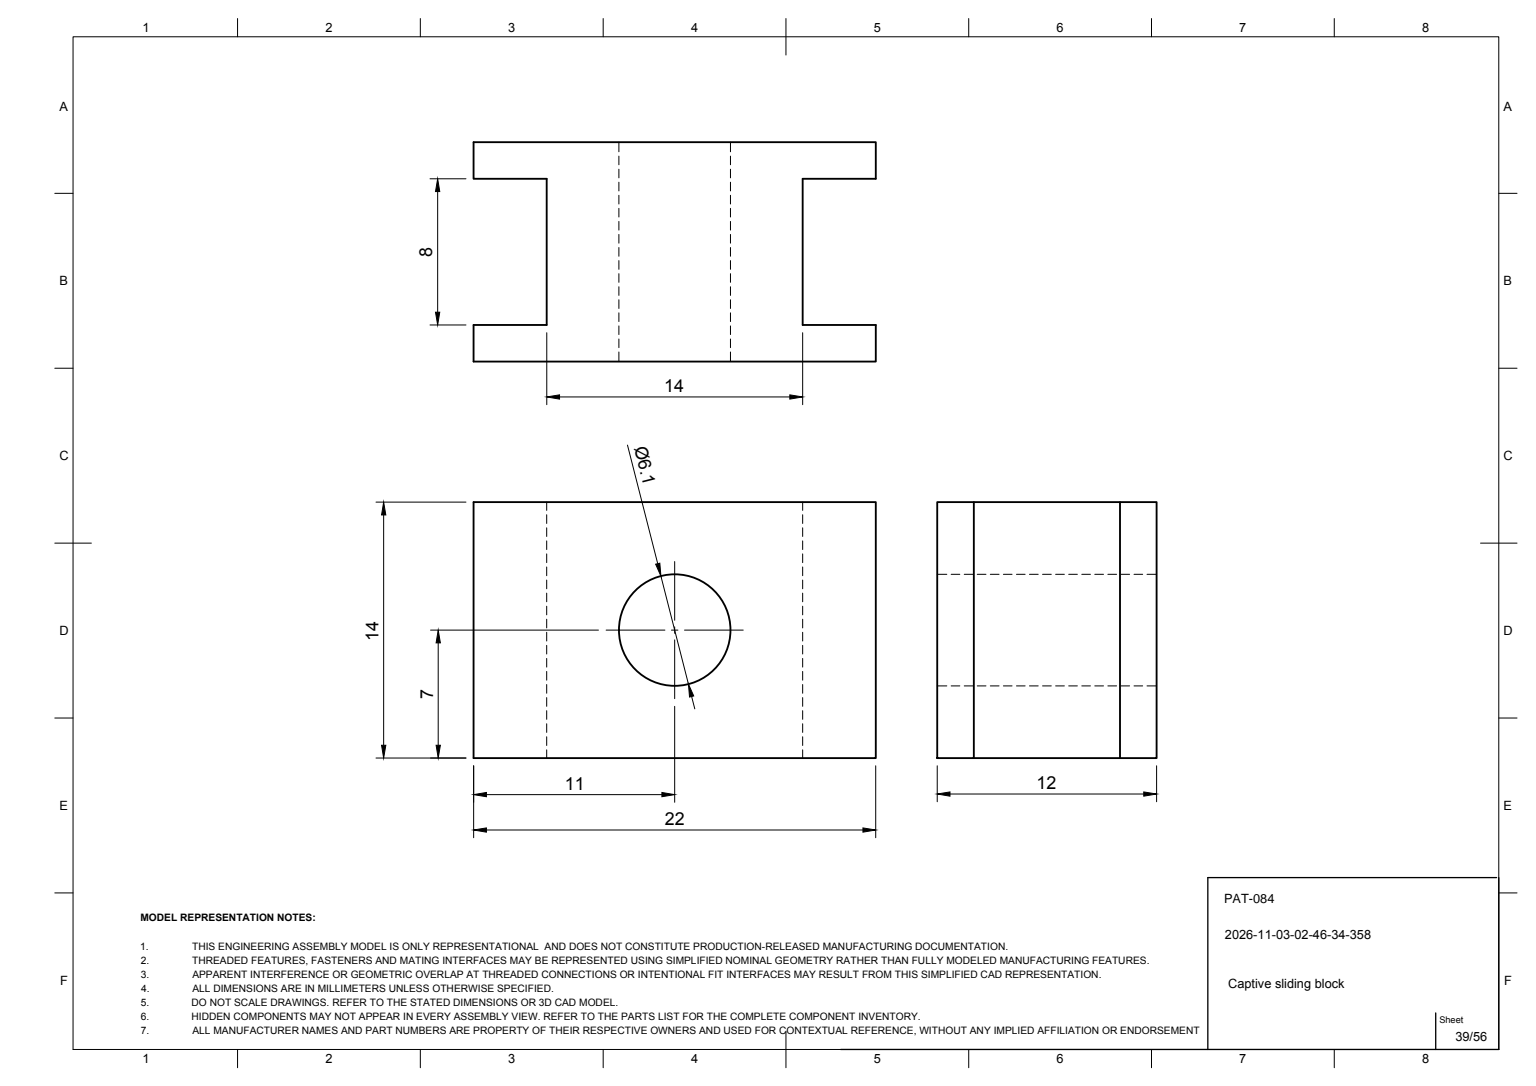
ISO-10303-21;
HEADER;
/* Generated by software containing ST-Developer
 * from STEP Tools, Inc. (www.steptools.com) 
 */

FILE_DESCRIPTION(
/* description */ ('Quick-return (Whitworth) mechanism'),
/* implementation_level */ '2;1');

FILE_NAME(
/* name */ 'Captive sliding block.step',
/* time_stamp */ '2026-10-28T03:25:57-07:00',
/* author */ (''),
/* organization */ (''),
/* preprocessor_version */ 'ST-DEVELOPER v20.2',
/* originating_system */ 'Autodesk Translation Framework v15.17.0.0',
/* authorisation */ '');

FILE_SCHEMA (('AUTOMOTIVE_DESIGN { 1 0 10303 214 3 1 1 }'));
ENDSEC;

DATA;
#10=MECHANICAL_DESIGN_GEOMETRIC_PRESENTATION_REPRESENTATION('',(#528),#14878);
#432=SHAPE_REPRESENTATION_RELATIONSHIP('SRR','None',#15104,#476);
#476=ADVANCED_BREP_SHAPE_REPRESENTATION('',(#579),#14861);
#528=STYLED_ITEM('',(#15385),#579);
#579=MANIFOLD_SOLID_BREP('Body1',#7883);
#747=FACE_BOUND('',#2004,.T.);
#748=FACE_BOUND('',#2010,.T.);
#948=PLANE('',#9095);
#949=PLANE('',#9096);
#950=PLANE('',#9097);
#951=PLANE('',#9098);
#952=PLANE('',#9099);
#953=PLANE('',#9100);
#954=PLANE('',#9101);
#955=PLANE('',#9102);
#956=PLANE('',#9103);
#957=PLANE('',#9104);
#958=PLANE('',#9105);
#959=PLANE('',#9106);
#960=PLANE('',#9107);
#961=PLANE('',#9108);
#1376=FACE_OUTER_BOUND('',#1998,.T.);
#1377=FACE_OUTER_BOUND('',#1999,.T.);
#1378=FACE_OUTER_BOUND('',#2000,.T.);
#1379=FACE_OUTER_BOUND('',#2001,.T.);
#1380=FACE_OUTER_BOUND('',#2002,.T.);
#1381=FACE_OUTER_BOUND('',#2003,.T.);
#1382=FACE_OUTER_BOUND('',#2005,.T.);
#1383=FACE_OUTER_BOUND('',#2006,.T.);
#1384=FACE_OUTER_BOUND('',#2007,.T.);
#1385=FACE_OUTER_BOUND('',#2008,.T.);
#1386=FACE_OUTER_BOUND('',#2009,.T.);
#1387=FACE_OUTER_BOUND('',#2011,.T.);
#1388=FACE_OUTER_BOUND('',#2012,.T.);
#1389=FACE_OUTER_BOUND('',#2013,.T.);
#1390=FACE_OUTER_BOUND('',#2014,.T.);
#1998=EDGE_LOOP('',(#6598,#6599,#6600,#6601));
#1999=EDGE_LOOP('',(#6602,#6603,#6604,#6605));
#2000=EDGE_LOOP('',(#6606,#6607,#6608,#6609));
#2001=EDGE_LOOP('',(#6610,#6611,#6612,#6613));
#2002=EDGE_LOOP('',(#6614,#6615,#6616,#6617));
#2003=EDGE_LOOP('',(#6618,#6619,#6620,#6621));
#2004=EDGE_LOOP('',(#6622));
#2005=EDGE_LOOP('',(#6623,#6624,#6625,#6626));
#2006=EDGE_LOOP('',(#6627,#6628,#6629,#6630));
#2007=EDGE_LOOP('',(#6631,#6632,#6633,#6634));
#2008=EDGE_LOOP('',(#6635,#6636,#6637,#6638));
#2009=EDGE_LOOP('',(#6639,#6640,#6641,#6642));
#2010=EDGE_LOOP('',(#6643));
#2011=EDGE_LOOP('',(#6644,#6645,#6646,#6647,#6648,#6649,#6650,#6651,#6652,
#6653,#6654,#6655));
#2012=EDGE_LOOP('',(#6656,#6657,#6658,#6659));
#2013=EDGE_LOOP('',(#6660,#6661,#6662,#6663,#6664,#6665,#6666,#6667,#6668,
#6669,#6670,#6671));
#2014=EDGE_LOOP('',(#6672,#6673,#6674,#6675));
#2465=LINE('',#14040,#2988);
#2466=LINE('',#14045,#2989);
#2467=LINE('',#14047,#2990);
#2468=LINE('',#14049,#2991);
#2469=LINE('',#14050,#2992);
#2470=LINE('',#14054,#2993);
#2471=LINE('',#14056,#2994);
#2472=LINE('',#14058,#2995);
#2473=LINE('',#14059,#2996);
#2474=LINE('',#14062,#2997);
#2475=LINE('',#14064,#2998);
#2476=LINE('',#14065,#2999);
#2477=LINE('',#14068,#3000);
#2478=LINE('',#14070,#3001);
#2479=LINE('',#14071,#3002);
#2480=LINE('',#14073,#3003);
#2481=LINE('',#14074,#3004);
#2482=LINE('',#14078,#3005);
#2483=LINE('',#14080,#3006);
#2484=LINE('',#14082,#3007);
#2485=LINE('',#14083,#3008);
#2486=LINE('',#14087,#3009);
#2487=LINE('',#14089,#3010);
#2488=LINE('',#14091,#3011);
#2489=LINE('',#14092,#3012);
#2490=LINE('',#14096,#3013);
#2491=LINE('',#14097,#3014);
#2492=LINE('',#14098,#3015);
#2493=LINE('',#14102,#3016);
#2494=LINE('',#14103,#3017);
#2495=LINE('',#14104,#3018);
#2496=LINE('',#14106,#3019);
#2497=LINE('',#14107,#3020);
#2498=LINE('',#14109,#3021);
#2499=LINE('',#14110,#3022);
#2500=LINE('',#14112,#3023);
#2501=LINE('',#14114,#3024);
#2988=VECTOR('',#11112,0.305);
#2989=VECTOR('',#11117,1.);
#2990=VECTOR('',#11118,1.);
#2991=VECTOR('',#11119,1.);
#2992=VECTOR('',#11120,1.);
#2993=VECTOR('',#11123,1.);
#2994=VECTOR('',#11124,1.);
#2995=VECTOR('',#11125,1.);
#2996=VECTOR('',#11126,1.);
#2997=VECTOR('',#11129,1.);
#2998=VECTOR('',#11130,1.);
#2999=VECTOR('',#11131,1.);
#3000=VECTOR('',#11134,1.);
#3001=VECTOR('',#11135,1.);
#3002=VECTOR('',#11136,1.);
#3003=VECTOR('',#11139,1.);
#3004=VECTOR('',#11140,1.);
#3005=VECTOR('',#11143,1.);
#3006=VECTOR('',#11144,1.);
#3007=VECTOR('',#11145,1.);
#3008=VECTOR('',#11146,1.);
#3009=VECTOR('',#11149,1.);
#3010=VECTOR('',#11150,1.);
#3011=VECTOR('',#11151,1.);
#3012=VECTOR('',#11152,1.);
#3013=VECTOR('',#11155,1.);
#3014=VECTOR('',#11156,1.);
#3015=VECTOR('',#11157,1.);
#3016=VECTOR('',#11160,1.);
#3017=VECTOR('',#11161,1.);
#3018=VECTOR('',#11162,1.);
#3019=VECTOR('',#11165,1.);
#3020=VECTOR('',#11166,1.);
#3021=VECTOR('',#11169,1.);
#3022=VECTOR('',#11170,1.);
#3023=VECTOR('',#11173,1.);
#3024=VECTOR('',#11176,1.);
#3553=CIRCLE('',#9093,0.305);
#3554=CIRCLE('',#9094,0.305);
#4086=VERTEX_POINT('',#14037);
#4087=VERTEX_POINT('',#14039);
#4088=VERTEX_POINT('',#14043);
#4089=VERTEX_POINT('',#14044);
#4090=VERTEX_POINT('',#14046);
#4091=VERTEX_POINT('',#14048);
#4092=VERTEX_POINT('',#14052);
#4093=VERTEX_POINT('',#14053);
#4094=VERTEX_POINT('',#14055);
#4095=VERTEX_POINT('',#14057);
#4096=VERTEX_POINT('',#14061);
#4097=VERTEX_POINT('',#14063);
#4098=VERTEX_POINT('',#14067);
#4099=VERTEX_POINT('',#14069);
#4100=VERTEX_POINT('',#14076);
#4101=VERTEX_POINT('',#14077);
#4102=VERTEX_POINT('',#14079);
#4103=VERTEX_POINT('',#14081);
#4104=VERTEX_POINT('',#14085);
#4105=VERTEX_POINT('',#14086);
#4106=VERTEX_POINT('',#14088);
#4107=VERTEX_POINT('',#14090);
#4108=VERTEX_POINT('',#14094);
#4109=VERTEX_POINT('',#14095);
#4110=VERTEX_POINT('',#14100);
#4111=VERTEX_POINT('',#14101);
#4956=EDGE_CURVE('',#4086,#4086,#3553,.T.);
#4957=EDGE_CURVE('',#4086,#4087,#2465,.T.);
#4958=EDGE_CURVE('',#4087,#4087,#3554,.T.);
#4959=EDGE_CURVE('',#4088,#4089,#2466,.T.);
#4960=EDGE_CURVE('',#4090,#4089,#2467,.T.);
#4961=EDGE_CURVE('',#4091,#4090,#2468,.T.);
#4962=EDGE_CURVE('',#4088,#4091,#2469,.T.);
#4963=EDGE_CURVE('',#4092,#4093,#2470,.T.);
#4964=EDGE_CURVE('',#4094,#4093,#2471,.T.);
#4965=EDGE_CURVE('',#4095,#4094,#2472,.T.);
#4966=EDGE_CURVE('',#4092,#4095,#2473,.T.);
#4967=EDGE_CURVE('',#4090,#4096,#2474,.T.);
#4968=EDGE_CURVE('',#4097,#4096,#2475,.T.);
#4969=EDGE_CURVE('',#4091,#4097,#2476,.T.);
#4970=EDGE_CURVE('',#4094,#4098,#2477,.T.);
#4971=EDGE_CURVE('',#4099,#4098,#2478,.T.);
#4972=EDGE_CURVE('',#4095,#4099,#2479,.T.);
#4973=EDGE_CURVE('',#4098,#4097,#2480,.T.);
#4974=EDGE_CURVE('',#4096,#4099,#2481,.T.);
#4975=EDGE_CURVE('',#4100,#4101,#2482,.T.);
#4976=EDGE_CURVE('',#4100,#4102,#2483,.T.);
#4977=EDGE_CURVE('',#4102,#4103,#2484,.T.);
#4978=EDGE_CURVE('',#4103,#4101,#2485,.T.);
#4979=EDGE_CURVE('',#4104,#4105,#2486,.T.);
#4980=EDGE_CURVE('',#4104,#4106,#2487,.T.);
#4981=EDGE_CURVE('',#4106,#4107,#2488,.T.);
#4982=EDGE_CURVE('',#4107,#4105,#2489,.T.);
#4983=EDGE_CURVE('',#4108,#4109,#2490,.T.);
#4984=EDGE_CURVE('',#4109,#4107,#2491,.T.);
#4985=EDGE_CURVE('',#4108,#4106,#2492,.T.);
#4986=EDGE_CURVE('',#4110,#4111,#2493,.T.);
#4987=EDGE_CURVE('',#4111,#4103,#2494,.T.);
#4988=EDGE_CURVE('',#4110,#4102,#2495,.T.);
#4989=EDGE_CURVE('',#4109,#4110,#2496,.T.);
#4990=EDGE_CURVE('',#4111,#4108,#2497,.T.);
#4991=EDGE_CURVE('',#4100,#4092,#2498,.T.);
#4992=EDGE_CURVE('',#4105,#4089,#2499,.T.);
#4993=EDGE_CURVE('',#4104,#4088,#2500,.T.);
#4994=EDGE_CURVE('',#4101,#4093,#2501,.T.);
#6598=ORIENTED_EDGE('',*,*,#4956,.F.);
#6599=ORIENTED_EDGE('',*,*,#4957,.T.);
#6600=ORIENTED_EDGE('',*,*,#4958,.F.);
#6601=ORIENTED_EDGE('',*,*,#4957,.F.);
#6602=ORIENTED_EDGE('',*,*,#4959,.T.);
#6603=ORIENTED_EDGE('',*,*,#4960,.F.);
#6604=ORIENTED_EDGE('',*,*,#4961,.F.);
#6605=ORIENTED_EDGE('',*,*,#4962,.F.);
#6606=ORIENTED_EDGE('',*,*,#4963,.T.);
#6607=ORIENTED_EDGE('',*,*,#4964,.F.);
#6608=ORIENTED_EDGE('',*,*,#4965,.F.);
#6609=ORIENTED_EDGE('',*,*,#4966,.F.);
#6610=ORIENTED_EDGE('',*,*,#4961,.T.);
#6611=ORIENTED_EDGE('',*,*,#4967,.T.);
#6612=ORIENTED_EDGE('',*,*,#4968,.F.);
#6613=ORIENTED_EDGE('',*,*,#4969,.F.);
#6614=ORIENTED_EDGE('',*,*,#4965,.T.);
#6615=ORIENTED_EDGE('',*,*,#4970,.T.);
#6616=ORIENTED_EDGE('',*,*,#4971,.F.);
#6617=ORIENTED_EDGE('',*,*,#4972,.F.);
#6618=ORIENTED_EDGE('',*,*,#4971,.T.);
#6619=ORIENTED_EDGE('',*,*,#4973,.T.);
#6620=ORIENTED_EDGE('',*,*,#4968,.T.);
#6621=ORIENTED_EDGE('',*,*,#4974,.T.);
#6622=ORIENTED_EDGE('',*,*,#4958,.T.);
#6623=ORIENTED_EDGE('',*,*,#4975,.F.);
#6624=ORIENTED_EDGE('',*,*,#4976,.T.);
#6625=ORIENTED_EDGE('',*,*,#4977,.T.);
#6626=ORIENTED_EDGE('',*,*,#4978,.T.);
#6627=ORIENTED_EDGE('',*,*,#4979,.F.);
#6628=ORIENTED_EDGE('',*,*,#4980,.T.);
#6629=ORIENTED_EDGE('',*,*,#4981,.T.);
#6630=ORIENTED_EDGE('',*,*,#4982,.T.);
#6631=ORIENTED_EDGE('',*,*,#4983,.T.);
#6632=ORIENTED_EDGE('',*,*,#4984,.T.);
#6633=ORIENTED_EDGE('',*,*,#4981,.F.);
#6634=ORIENTED_EDGE('',*,*,#4985,.F.);
#6635=ORIENTED_EDGE('',*,*,#4986,.T.);
#6636=ORIENTED_EDGE('',*,*,#4987,.T.);
#6637=ORIENTED_EDGE('',*,*,#4977,.F.);
#6638=ORIENTED_EDGE('',*,*,#4988,.F.);
#6639=ORIENTED_EDGE('',*,*,#4986,.F.);
#6640=ORIENTED_EDGE('',*,*,#4989,.F.);
#6641=ORIENTED_EDGE('',*,*,#4983,.F.);
#6642=ORIENTED_EDGE('',*,*,#4990,.F.);
#6643=ORIENTED_EDGE('',*,*,#4956,.T.);
#6644=ORIENTED_EDGE('',*,*,#4991,.T.);
#6645=ORIENTED_EDGE('',*,*,#4966,.T.);
#6646=ORIENTED_EDGE('',*,*,#4972,.T.);
#6647=ORIENTED_EDGE('',*,*,#4974,.F.);
#6648=ORIENTED_EDGE('',*,*,#4967,.F.);
#6649=ORIENTED_EDGE('',*,*,#4960,.T.);
#6650=ORIENTED_EDGE('',*,*,#4992,.F.);
#6651=ORIENTED_EDGE('',*,*,#4982,.F.);
#6652=ORIENTED_EDGE('',*,*,#4984,.F.);
#6653=ORIENTED_EDGE('',*,*,#4989,.T.);
#6654=ORIENTED_EDGE('',*,*,#4988,.T.);
#6655=ORIENTED_EDGE('',*,*,#4976,.F.);
#6656=ORIENTED_EDGE('',*,*,#4979,.T.);
#6657=ORIENTED_EDGE('',*,*,#4992,.T.);
#6658=ORIENTED_EDGE('',*,*,#4959,.F.);
#6659=ORIENTED_EDGE('',*,*,#4993,.F.);
#6660=ORIENTED_EDGE('',*,*,#4993,.T.);
#6661=ORIENTED_EDGE('',*,*,#4962,.T.);
#6662=ORIENTED_EDGE('',*,*,#4969,.T.);
#6663=ORIENTED_EDGE('',*,*,#4973,.F.);
#6664=ORIENTED_EDGE('',*,*,#4970,.F.);
#6665=ORIENTED_EDGE('',*,*,#4964,.T.);
#6666=ORIENTED_EDGE('',*,*,#4994,.F.);
#6667=ORIENTED_EDGE('',*,*,#4978,.F.);
#6668=ORIENTED_EDGE('',*,*,#4987,.F.);
#6669=ORIENTED_EDGE('',*,*,#4990,.T.);
#6670=ORIENTED_EDGE('',*,*,#4985,.T.);
#6671=ORIENTED_EDGE('',*,*,#4980,.F.);
#6672=ORIENTED_EDGE('',*,*,#4975,.T.);
#6673=ORIENTED_EDGE('',*,*,#4994,.T.);
#6674=ORIENTED_EDGE('',*,*,#4963,.F.);
#6675=ORIENTED_EDGE('',*,*,#4991,.F.);
#7346=CYLINDRICAL_SURFACE('',#9092,0.305);
#7707=ADVANCED_FACE('',(#1376),#7346,.F.);
#7708=ADVANCED_FACE('',(#1377),#948,.F.);
#7709=ADVANCED_FACE('',(#1378),#949,.F.);
#7710=ADVANCED_FACE('',(#1379),#950,.T.);
#7711=ADVANCED_FACE('',(#1380),#951,.T.);
#7712=ADVANCED_FACE('',(#1381,#747),#952,.T.);
#7713=ADVANCED_FACE('',(#1382),#953,.T.);
#7714=ADVANCED_FACE('',(#1383),#954,.T.);
#7715=ADVANCED_FACE('',(#1384),#955,.T.);
#7716=ADVANCED_FACE('',(#1385),#956,.T.);
#7717=ADVANCED_FACE('',(#1386,#748),#957,.F.);
#7718=ADVANCED_FACE('',(#1387),#958,.T.);
#7719=ADVANCED_FACE('',(#1388),#959,.T.);
#7720=ADVANCED_FACE('',(#1389),#960,.T.);
#7721=ADVANCED_FACE('',(#1390),#961,.T.);
#7883=CLOSED_SHELL('',(#7707,#7708,#7709,#7710,#7711,#7712,#7713,#7714,
#7715,#7716,#7717,#7718,#7719,#7720,#7721));
#9091=AXIS2_PLACEMENT_3D('',#14035,#11106,#11107);
#9092=AXIS2_PLACEMENT_3D('',#14036,#11108,#11109);
#9093=AXIS2_PLACEMENT_3D('',#14038,#11110,#11111);
#9094=AXIS2_PLACEMENT_3D('',#14041,#11113,#11114);
#9095=AXIS2_PLACEMENT_3D('',#14042,#11115,#11116);
#9096=AXIS2_PLACEMENT_3D('',#14051,#11121,#11122);
#9097=AXIS2_PLACEMENT_3D('',#14060,#11127,#11128);
#9098=AXIS2_PLACEMENT_3D('',#14066,#11132,#11133);
#9099=AXIS2_PLACEMENT_3D('',#14072,#11137,#11138);
#9100=AXIS2_PLACEMENT_3D('',#14075,#11141,#11142);
#9101=AXIS2_PLACEMENT_3D('',#14084,#11147,#11148);
#9102=AXIS2_PLACEMENT_3D('',#14093,#11153,#11154);
#9103=AXIS2_PLACEMENT_3D('',#14099,#11158,#11159);
#9104=AXIS2_PLACEMENT_3D('',#14105,#11163,#11164);
#9105=AXIS2_PLACEMENT_3D('',#14108,#11167,#11168);
#9106=AXIS2_PLACEMENT_3D('',#14111,#11171,#11172);
#9107=AXIS2_PLACEMENT_3D('',#14113,#11174,#11175);
#9108=AXIS2_PLACEMENT_3D('',#14115,#11177,#11178);
#11106=DIRECTION('axis',(0.,0.,1.));
#11107=DIRECTION('refdir',(1.,0.,0.));
#11108=DIRECTION('center_axis',(0.,0.,1.));
#11109=DIRECTION('ref_axis',(1.,0.,0.));
#11110=DIRECTION('center_axis',(0.,0.,1.));
#11111=DIRECTION('ref_axis',(1.,0.,0.));
#11112=DIRECTION('',(0.,0.,1.));
#11113=DIRECTION('center_axis',(0.,0.,-1.));
#11114=DIRECTION('ref_axis',(1.,0.,0.));
#11115=DIRECTION('center_axis',(0.,0.,1.));
#11116=DIRECTION('ref_axis',(1.,0.,0.));
#11117=DIRECTION('',(0.,1.,0.));
#11118=DIRECTION('',(-1.,0.,0.));
#11119=DIRECTION('',(0.,1.,0.));
#11120=DIRECTION('',(1.,0.,0.));
#11121=DIRECTION('center_axis',(0.,0.,1.));
#11122=DIRECTION('ref_axis',(1.,0.,0.));
#11123=DIRECTION('',(0.,-1.,0.));
#11124=DIRECTION('',(1.,0.,0.));
#11125=DIRECTION('',(0.,-1.,0.));
#11126=DIRECTION('',(-1.,0.,0.));
#11127=DIRECTION('center_axis',(1.,0.,0.));
#11128=DIRECTION('ref_axis',(0.,1.,0.));
#11129=DIRECTION('',(0.,0.,1.));
#11130=DIRECTION('',(0.,1.,0.));
#11131=DIRECTION('',(0.,0.,1.));
#11132=DIRECTION('center_axis',(-1.,0.,0.));
#11133=DIRECTION('ref_axis',(0.,-1.,0.));
#11134=DIRECTION('',(0.,0.,1.));
#11135=DIRECTION('',(0.,-1.,0.));
#11136=DIRECTION('',(0.,0.,1.));
#11137=DIRECTION('center_axis',(0.,0.,1.));
#11138=DIRECTION('ref_axis',(1.,0.,0.));
#11139=DIRECTION('',(1.,0.,0.));
#11140=DIRECTION('',(-1.,0.,0.));
#11141=DIRECTION('center_axis',(0.,0.,1.));
#11142=DIRECTION('ref_axis',(1.,0.,0.));
#11143=DIRECTION('',(0.,-1.,0.));
#11144=DIRECTION('',(-1.,0.,0.));
#11145=DIRECTION('',(0.,-1.,0.));
#11146=DIRECTION('',(1.,0.,0.));
#11147=DIRECTION('center_axis',(0.,0.,1.));
#11148=DIRECTION('ref_axis',(1.,0.,0.));
#11149=DIRECTION('',(0.,1.,0.));
#11150=DIRECTION('',(1.,0.,0.));
#11151=DIRECTION('',(0.,1.,0.));
#11152=DIRECTION('',(-1.,0.,0.));
#11153=DIRECTION('center_axis',(1.,0.,0.));
#11154=DIRECTION('ref_axis',(0.,1.,0.));
#11155=DIRECTION('',(0.,1.,0.));
#11156=DIRECTION('',(0.,0.,1.));
#11157=DIRECTION('',(0.,0.,1.));
#11158=DIRECTION('center_axis',(-1.,0.,0.));
#11159=DIRECTION('ref_axis',(0.,-1.,0.));
#11160=DIRECTION('',(0.,-1.,0.));
#11161=DIRECTION('',(0.,0.,1.));
#11162=DIRECTION('',(0.,0.,1.));
#11163=DIRECTION('center_axis',(0.,0.,1.));
#11164=DIRECTION('ref_axis',(1.,0.,0.));
#11165=DIRECTION('',(-1.,0.,0.));
#11166=DIRECTION('',(1.,0.,0.));
#11167=DIRECTION('center_axis',(0.,1.,0.));
#11168=DIRECTION('ref_axis',(-1.,0.,0.));
#11169=DIRECTION('',(0.,0.,1.));
#11170=DIRECTION('',(0.,0.,1.));
#11171=DIRECTION('center_axis',(1.,0.,0.));
#11172=DIRECTION('ref_axis',(0.,1.,0.));
#11173=DIRECTION('',(0.,0.,1.));
#11174=DIRECTION('center_axis',(0.,-1.,0.));
#11175=DIRECTION('ref_axis',(1.,0.,0.));
#11176=DIRECTION('',(0.,0.,1.));
#11177=DIRECTION('center_axis',(-1.,0.,0.));
#11178=DIRECTION('ref_axis',(0.,-1.,0.));
#14035=CARTESIAN_POINT('',(0.,0.,0.));
#14036=CARTESIAN_POINT('Origin',(0.,9.,6.1));
#14037=CARTESIAN_POINT('',(-0.305,9.,6.2));
#14038=CARTESIAN_POINT('Origin',(0.,9.,6.2));
#14039=CARTESIAN_POINT('',(-0.305,9.,7.4));
#14040=CARTESIAN_POINT('',(-0.305,9.,6.1));
#14041=CARTESIAN_POINT('Origin',(0.,9.,7.4));
#14042=CARTESIAN_POINT('Origin',(0.,9.,7.2));
#14043=CARTESIAN_POINT('',(0.7,8.3,7.2));
#14044=CARTESIAN_POINT('',(0.7,9.7,7.2));
#14045=CARTESIAN_POINT('',(0.7,8.3,7.2));
#14046=CARTESIAN_POINT('',(1.1,9.7,7.2));
#14047=CARTESIAN_POINT('',(1.1,9.7,7.2));
#14048=CARTESIAN_POINT('',(1.1,8.3,7.2));
#14049=CARTESIAN_POINT('',(1.1,8.3,7.2));
#14050=CARTESIAN_POINT('',(-1.1,8.3,7.2));
#14051=CARTESIAN_POINT('Origin',(0.,9.,7.2));
#14052=CARTESIAN_POINT('',(-0.7,9.7,7.2));
#14053=CARTESIAN_POINT('',(-0.7,8.3,7.2));
#14054=CARTESIAN_POINT('',(-0.7,9.7,7.2));
#14055=CARTESIAN_POINT('',(-1.1,8.3,7.2));
#14056=CARTESIAN_POINT('',(-1.1,8.3,7.2));
#14057=CARTESIAN_POINT('',(-1.1,9.7,7.2));
#14058=CARTESIAN_POINT('',(-1.1,9.7,7.2));
#14059=CARTESIAN_POINT('',(1.1,9.7,7.2));
#14060=CARTESIAN_POINT('Origin',(1.1,8.3,7.2));
#14061=CARTESIAN_POINT('',(1.1,9.7,7.4));
#14062=CARTESIAN_POINT('',(1.1,9.7,7.2));
#14063=CARTESIAN_POINT('',(1.1,8.3,7.4));
#14064=CARTESIAN_POINT('',(1.1,8.3,7.4));
#14065=CARTESIAN_POINT('',(1.1,8.3,7.2));
#14066=CARTESIAN_POINT('Origin',(-1.1,9.7,7.2));
#14067=CARTESIAN_POINT('',(-1.1,8.3,7.4));
#14068=CARTESIAN_POINT('',(-1.1,8.3,7.2));
#14069=CARTESIAN_POINT('',(-1.1,9.7,7.4));
#14070=CARTESIAN_POINT('',(-1.1,9.7,7.4));
#14071=CARTESIAN_POINT('',(-1.1,9.7,7.2));
#14072=CARTESIAN_POINT('Origin',(0.,9.,7.4));
#14073=CARTESIAN_POINT('',(-1.1,8.3,7.4));
#14074=CARTESIAN_POINT('',(1.1,9.7,7.4));
#14075=CARTESIAN_POINT('Origin',(0.,9.,6.4));
#14076=CARTESIAN_POINT('',(-0.7,9.7,6.4));
#14077=CARTESIAN_POINT('',(-0.7,8.3,6.4));
#14078=CARTESIAN_POINT('',(-0.7,9.7,6.4));
#14079=CARTESIAN_POINT('',(-1.1,9.7,6.4));
#14080=CARTESIAN_POINT('',(1.1,9.7,6.4));
#14081=CARTESIAN_POINT('',(-1.1,8.3,6.4));
#14082=CARTESIAN_POINT('',(-1.1,9.7,6.4));
#14083=CARTESIAN_POINT('',(-1.1,8.3,6.4));
#14084=CARTESIAN_POINT('Origin',(0.,9.,6.4));
#14085=CARTESIAN_POINT('',(0.7,8.3,6.4));
#14086=CARTESIAN_POINT('',(0.7,9.7,6.4));
#14087=CARTESIAN_POINT('',(0.7,8.3,6.4));
#14088=CARTESIAN_POINT('',(1.1,8.3,6.4));
#14089=CARTESIAN_POINT('',(-1.1,8.3,6.4));
#14090=CARTESIAN_POINT('',(1.1,9.7,6.4));
#14091=CARTESIAN_POINT('',(1.1,8.3,6.4));
#14092=CARTESIAN_POINT('',(1.1,9.7,6.4));
#14093=CARTESIAN_POINT('Origin',(1.1,8.3,6.2));
#14094=CARTESIAN_POINT('',(1.1,8.3,6.2));
#14095=CARTESIAN_POINT('',(1.1,9.7,6.2));
#14096=CARTESIAN_POINT('',(1.1,8.3,6.2));
#14097=CARTESIAN_POINT('',(1.1,9.7,6.2));
#14098=CARTESIAN_POINT('',(1.1,8.3,6.2));
#14099=CARTESIAN_POINT('Origin',(-1.1,9.7,6.2));
#14100=CARTESIAN_POINT('',(-1.1,9.7,6.2));
#14101=CARTESIAN_POINT('',(-1.1,8.3,6.2));
#14102=CARTESIAN_POINT('',(-1.1,9.7,6.2));
#14103=CARTESIAN_POINT('',(-1.1,8.3,6.2));
#14104=CARTESIAN_POINT('',(-1.1,9.7,6.2));
#14105=CARTESIAN_POINT('Origin',(0.,9.,6.2));
#14106=CARTESIAN_POINT('',(1.1,9.7,6.2));
#14107=CARTESIAN_POINT('',(-1.1,8.3,6.2));
#14108=CARTESIAN_POINT('Origin',(0.7,9.7,6.4));
#14109=CARTESIAN_POINT('',(-0.7,9.7,6.4));
#14110=CARTESIAN_POINT('',(0.7,9.7,6.4));
#14111=CARTESIAN_POINT('Origin',(0.7,8.3,6.4));
#14112=CARTESIAN_POINT('',(0.7,8.3,6.4));
#14113=CARTESIAN_POINT('Origin',(-0.7,8.3,6.4));
#14114=CARTESIAN_POINT('',(-0.7,8.3,6.4));
#14115=CARTESIAN_POINT('Origin',(-0.7,9.7,6.4));
#14807=UNCERTAINTY_MEASURE_WITH_UNIT(LENGTH_MEASURE(0.001),#14879,
'DISTANCE_ACCURACY_VALUE',
'Maximum model space distance between geometric entities at asserted c
onnectivities');
#14824=UNCERTAINTY_MEASURE_WITH_UNIT(LENGTH_MEASURE(0.001),#14879,
'DISTANCE_ACCURACY_VALUE',
'Maximum model space distance between geometric entities at asserted c
onnectivities');
#14861=(
GEOMETRIC_REPRESENTATION_CONTEXT(3)
GLOBAL_UNCERTAINTY_ASSIGNED_CONTEXT((#14807))
GLOBAL_UNIT_ASSIGNED_CONTEXT((#14879,#14881,#14882))
REPRESENTATION_CONTEXT('','3D')
);
#14878=(
GEOMETRIC_REPRESENTATION_CONTEXT(3)
GLOBAL_UNCERTAINTY_ASSIGNED_CONTEXT((#14824))
GLOBAL_UNIT_ASSIGNED_CONTEXT((#14879,#14881,#14882))
REPRESENTATION_CONTEXT('','3D')
);
#14879=(
LENGTH_UNIT()
NAMED_UNIT(*)
SI_UNIT(.CENTI.,.METRE.)
);
#14881=(
NAMED_UNIT(*)
PLANE_ANGLE_UNIT()
SI_UNIT($,.RADIAN.)
);
#14882=(
NAMED_UNIT(*)
SI_UNIT($,.STERADIAN.)
SOLID_ANGLE_UNIT()
);
#14919=SHAPE_DEFINITION_REPRESENTATION(#14977,#15104);
#14977=PRODUCT_DEFINITION_SHAPE('',$,#15158);
#15104=SHAPE_REPRESENTATION('',(#9091),#14861);
#15121=PRODUCT_DEFINITION_CONTEXT('part definition',#15282,'design');
#15158=PRODUCT_DEFINITION('Captive sliding block',
'Captive sliding block',#15211,#15121);
#15211=PRODUCT_DEFINITION_FORMATION('',$,#15320);
#15282=APPLICATION_CONTEXT(
'Core Data for Automotive Mechanical Design Process');
#15283=PRODUCT_CONTEXT('part definition',#15282,'mechanical');
#15320=PRODUCT('Captive sliding block','Captive sliding block',
'Captive sliding block',(#15283));
#15379=COLOUR_RGB('Dark Blue',0.08,0.2,0.34);
#15380=FILL_AREA_STYLE_COLOUR('',#15379);
#15381=FILL_AREA_STYLE('',(#15380));
#15382=SURFACE_STYLE_FILL_AREA(#15381);
#15383=SURFACE_SIDE_STYLE('',(#15382));
#15384=SURFACE_STYLE_USAGE(.BOTH.,#15383);
#15385=PRESENTATION_STYLE_ASSIGNMENT((#15384));
ENDSEC;
END-ISO-10303-21;
